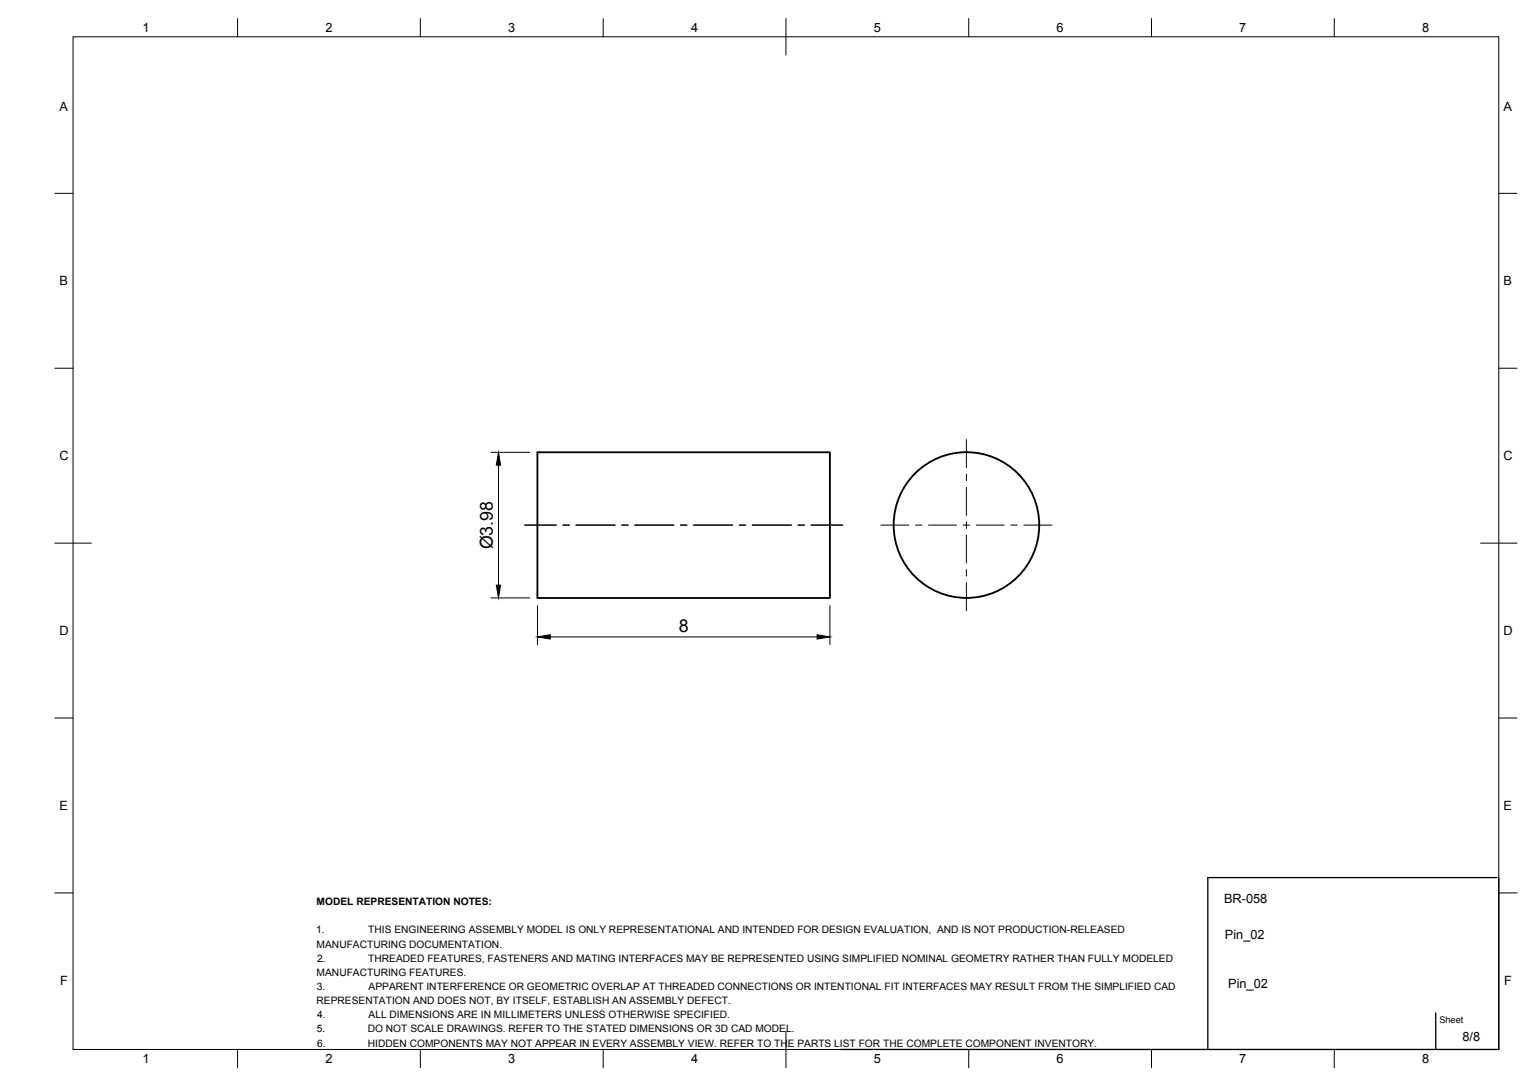
ISO-10303-21;
HEADER;
/* Generated by software containing ST-Developer
 * from STEP Tools, Inc. (www.steptools.com) 
 */

FILE_DESCRIPTION(
/* description */ (''),
/* implementation_level */ '2;1');

FILE_NAME(
/* name */ 'Pin_02.step',
/* time_stamp */ '2026-10-12T16:07:47-07:00',
/* author */ (''),
/* organization */ (''),
/* preprocessor_version */ 'ST-DEVELOPER v20.2',
/* originating_system */ 'Autodesk Translation Framework v15.15.0.0',
/* authorisation */ '');

FILE_SCHEMA (('AUTOMOTIVE_DESIGN { 1 0 10303 214 3 1 1 }'));
ENDSEC;

DATA;
#10=MECHANICAL_DESIGN_GEOMETRIC_PRESENTATION_REPRESENTATION('',(#99),#8779);
#85=SHAPE_REPRESENTATION_RELATIONSHIP('SRR','None',#8814,#92);
#92=ADVANCED_BREP_SHAPE_REPRESENTATION('',(#109),#8777);
#99=STYLED_ITEM('',(#8856),#109);
#109=MANIFOLD_SOLID_BREP('Body1',#5119);
#312=CIRCLE('',#5567,1.99137169252308);
#313=CIRCLE('',#5568,1.99137169252308);
#464=CYLINDRICAL_SURFACE('',#5566,1.99137169252308);
#689=FACE_OUTER_BOUND('',#1003,.T.);
#690=FACE_OUTER_BOUND('',#1004,.T.);
#691=FACE_OUTER_BOUND('',#1005,.T.);
#1003=EDGE_LOOP('',(#4458,#4459,#4460,#4461));
#1004=EDGE_LOOP('',(#4462));
#1005=EDGE_LOOP('',(#4463));
#1546=LINE('',#8523,#2031);
#2031=VECTOR('',#6916,1.99137169252308);
#2460=VERTEX_POINT('',#8520);
#2461=VERTEX_POINT('',#8522);
#3133=EDGE_CURVE('',#2460,#2460,#312,.T.);
#3134=EDGE_CURVE('',#2460,#2461,#1546,.T.);
#3135=EDGE_CURVE('',#2461,#2461,#313,.T.);
#4458=ORIENTED_EDGE('',*,*,#3133,.F.);
#4459=ORIENTED_EDGE('',*,*,#3134,.T.);
#4460=ORIENTED_EDGE('',*,*,#3135,.T.);
#4461=ORIENTED_EDGE('',*,*,#3134,.F.);
#4462=ORIENTED_EDGE('',*,*,#3133,.T.);
#4463=ORIENTED_EDGE('',*,*,#3135,.F.);
#4817=PLANE('',#5569);
#4818=PLANE('',#5570);
#5051=ADVANCED_FACE('',(#689),#464,.T.);
#5052=ADVANCED_FACE('',(#690),#4817,.T.);
#5053=ADVANCED_FACE('',(#691),#4818,.F.);
#5119=CLOSED_SHELL('',(#5051,#5052,#5053));
#5565=AXIS2_PLACEMENT_3D('',#8518,#6910,#6911);
#5566=AXIS2_PLACEMENT_3D('',#8519,#6912,#6913);
#5567=AXIS2_PLACEMENT_3D('',#8521,#6914,#6915);
#5568=AXIS2_PLACEMENT_3D('',#8524,#6917,#6918);
#5569=AXIS2_PLACEMENT_3D('',#8525,#6919,#6920);
#5570=AXIS2_PLACEMENT_3D('',#8526,#6921,#6922);
#6910=DIRECTION('axis',(0.,0.,1.));
#6911=DIRECTION('refdir',(1.,0.,0.));
#6912=DIRECTION('center_axis',(0.,-1.,0.));
#6913=DIRECTION('ref_axis',(1.,0.,0.));
#6914=DIRECTION('center_axis',(0.,-1.,0.));
#6915=DIRECTION('ref_axis',(1.,0.,0.));
#6916=DIRECTION('',(0.,1.,0.));
#6917=DIRECTION('center_axis',(0.,-1.,0.));
#6918=DIRECTION('ref_axis',(1.,0.,0.));
#6919=DIRECTION('center_axis',(0.,-1.,0.));
#6920=DIRECTION('ref_axis',(1.,0.,0.));
#6921=DIRECTION('center_axis',(0.,-1.,0.));
#6922=DIRECTION('ref_axis',(1.,0.,0.));
#8518=CARTESIAN_POINT('',(0.,0.,0.));
#8519=CARTESIAN_POINT('Origin',(0.,2.,48.6364583401654));
#8520=CARTESIAN_POINT('',(-1.99137169252308,-6.,48.6364583401654));
#8521=CARTESIAN_POINT('Origin',(0.,-6.,48.6364583401654));
#8522=CARTESIAN_POINT('',(-1.99137169252308,2.,48.6364583401654));
#8523=CARTESIAN_POINT('',(-1.99137169252308,2.,48.6364583401654));
#8524=CARTESIAN_POINT('Origin',(0.,2.,48.6364583401654));
#8525=CARTESIAN_POINT('Origin',(0.,-6.,48.6364583401654));
#8526=CARTESIAN_POINT('Origin',(0.,2.,48.6364583401654));
#8768=UNCERTAINTY_MEASURE_WITH_UNIT(LENGTH_MEASURE(0.01),#8780,
'DISTANCE_ACCURACY_VALUE',
'Maximum model space distance between geometric entities at asserted c
onnectivities');
#8770=UNCERTAINTY_MEASURE_WITH_UNIT(LENGTH_MEASURE(0.01),#8780,
'DISTANCE_ACCURACY_VALUE',
'Maximum model space distance between geometric entities at asserted c
onnectivities');
#8777=(
GEOMETRIC_REPRESENTATION_CONTEXT(3)
GLOBAL_UNCERTAINTY_ASSIGNED_CONTEXT((#8768))
GLOBAL_UNIT_ASSIGNED_CONTEXT((#8780,#8782,#8783))
REPRESENTATION_CONTEXT('','3D')
);
#8779=(
GEOMETRIC_REPRESENTATION_CONTEXT(3)
GLOBAL_UNCERTAINTY_ASSIGNED_CONTEXT((#8770))
GLOBAL_UNIT_ASSIGNED_CONTEXT((#8780,#8782,#8783))
REPRESENTATION_CONTEXT('','3D')
);
#8780=(
LENGTH_UNIT()
NAMED_UNIT(*)
SI_UNIT(.MILLI.,.METRE.)
);
#8782=(
NAMED_UNIT(*)
PLANE_ANGLE_UNIT()
SI_UNIT($,.RADIAN.)
);
#8783=(
NAMED_UNIT(*)
SI_UNIT($,.STERADIAN.)
SOLID_ANGLE_UNIT()
);
#8790=SHAPE_DEFINITION_REPRESENTATION(#8798,#8814);
#8798=PRODUCT_DEFINITION_SHAPE('',$,#8823);
#8814=SHAPE_REPRESENTATION('',(#5565),#8777);
#8816=PRODUCT_DEFINITION_CONTEXT('part definition',#8842,'design');
#8823=PRODUCT_DEFINITION('Pin_02','Pin_02',#8831,#8816);
#8831=PRODUCT_DEFINITION_FORMATION('',$,#8850);
#8842=APPLICATION_CONTEXT(
'Core Data for Automotive Mechanical Design Process');
#8843=PRODUCT_CONTEXT('part definition',#8842,'mechanical');
#8850=PRODUCT('Pin_02','Pin_02',$,(#8843));
#8856=PRESENTATION_STYLE_ASSIGNMENT((#8861));
#8861=SURFACE_STYLE_USAGE(.BOTH.,#8866);
#8866=SURFACE_SIDE_STYLE('',(#8871));
#8871=SURFACE_STYLE_FILL_AREA(#8876);
#8876=FILL_AREA_STYLE('Opaque(160,160,160)',(#8881));
#8881=FILL_AREA_STYLE_COLOUR('Opaque(160,160,160)',#8886);
#8886=COLOUR_RGB('Opaque(160,160,160)', 0.72549020, 0.75294118, 0.79215686);
ENDSEC;
END-ISO-10303-21;
